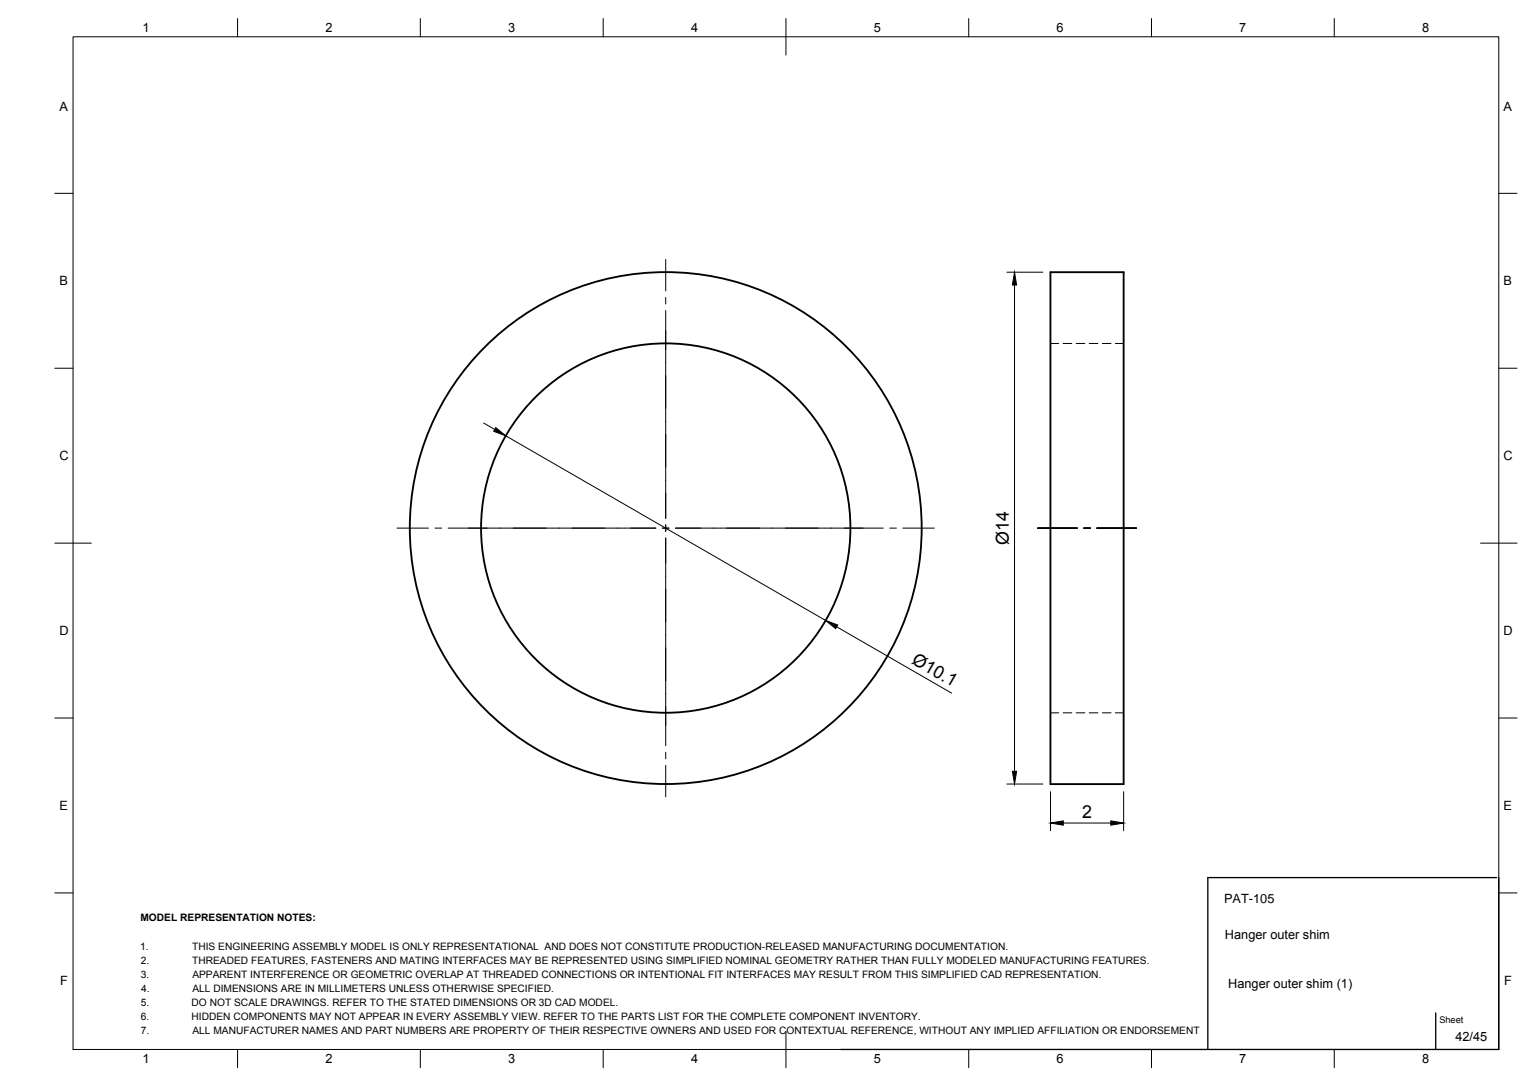
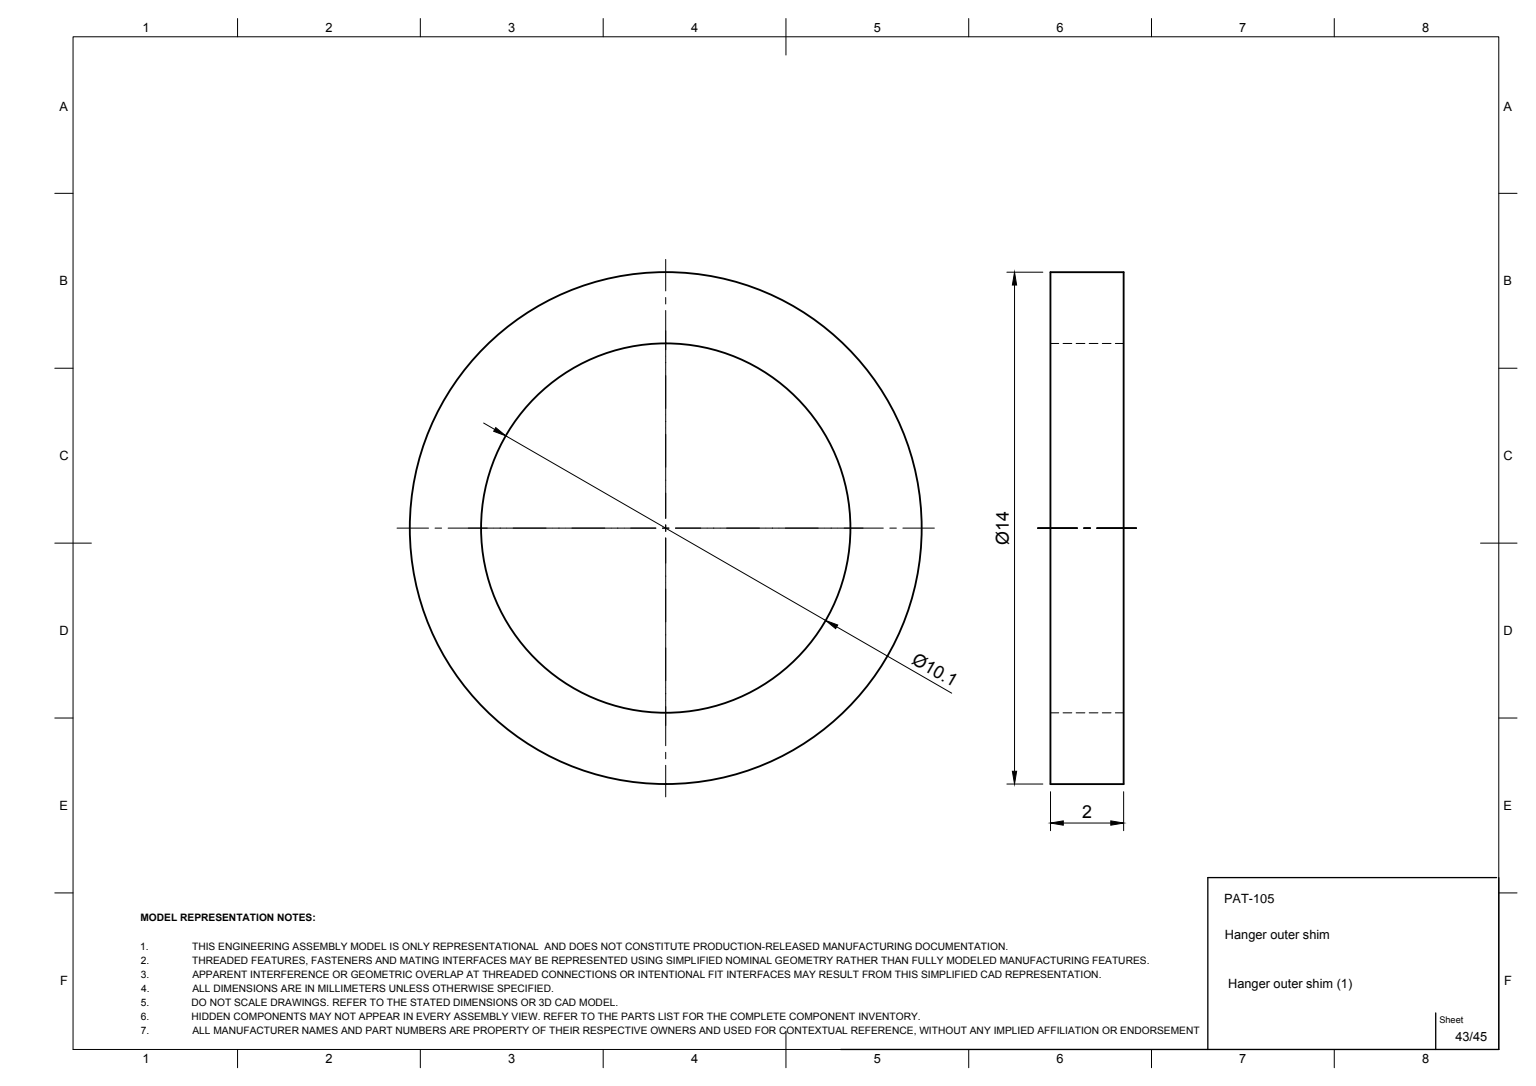
ISO-10303-21;
HEADER;
/* Generated by software containing ST-Developer
 * from STEP Tools, Inc. (www.steptools.com) 
 */

FILE_DESCRIPTION(
/* description */ ('Torque wrench calibration arm'),
/* implementation_level */ '2;1');

FILE_NAME(
/* name */ 'Hanger outer shim.step',
/* time_stamp */ '2026-10-28T03:24:52-07:00',
/* author */ (''),
/* organization */ (''),
/* preprocessor_version */ 'ST-DEVELOPER v20.2',
/* originating_system */ 'Autodesk Translation Framework v15.17.0.0',
/* authorisation */ '');

FILE_SCHEMA (('AUTOMOTIVE_DESIGN { 1 0 10303 214 3 1 1 }'));
ENDSEC;

DATA;
#10=MECHANICAL_DESIGN_GEOMETRIC_PRESENTATION_REPRESENTATION('',(#475),#12783);
#384=SHAPE_REPRESENTATION_RELATIONSHIP('SRR','None',#12969,#421);
#421=ADVANCED_BREP_SHAPE_REPRESENTATION('',(#527),#12778);
#475=STYLED_ITEM('',(#13205),#527);
#527=MANIFOLD_SOLID_BREP('Body1',#6546);
#643=FACE_BOUND('',#1748,.T.);
#644=FACE_BOUND('',#1750,.T.);
#856=PLANE('',#7744);
#857=PLANE('',#7745);
#1238=FACE_OUTER_BOUND('',#1745,.T.);
#1239=FACE_OUTER_BOUND('',#1746,.T.);
#1240=FACE_OUTER_BOUND('',#1747,.T.);
#1241=FACE_OUTER_BOUND('',#1749,.T.);
#1745=EDGE_LOOP('',(#5879,#5880,#5881,#5882));
#1746=EDGE_LOOP('',(#5883,#5884,#5885,#5886));
#1747=EDGE_LOOP('',(#5887));
#1748=EDGE_LOOP('',(#5888));
#1749=EDGE_LOOP('',(#5889));
#1750=EDGE_LOOP('',(#5890));
#2170=LINE('',#12562,#2585);
#2171=LINE('',#12568,#2586);
#2585=VECTOR('',#9754,0.505000000000003);
#2586=VECTOR('',#9761,0.700000000000003);
#2948=CIRCLE('',#7739,0.505000000000003);
#2949=CIRCLE('',#7740,0.505000000000003);
#2950=CIRCLE('',#7742,0.700000000000003);
#2951=CIRCLE('',#7743,0.700000000000003);
#3498=VERTEX_POINT('',#12559);
#3499=VERTEX_POINT('',#12561);
#3500=VERTEX_POINT('',#12565);
#3501=VERTEX_POINT('',#12567);
#4297=EDGE_CURVE('',#3498,#3498,#2948,.T.);
#4298=EDGE_CURVE('',#3498,#3499,#2170,.T.);
#4299=EDGE_CURVE('',#3499,#3499,#2949,.T.);
#4300=EDGE_CURVE('',#3500,#3500,#2950,.T.);
#4301=EDGE_CURVE('',#3500,#3501,#2171,.T.);
#4302=EDGE_CURVE('',#3501,#3501,#2951,.T.);
#5879=ORIENTED_EDGE('',*,*,#4297,.F.);
#5880=ORIENTED_EDGE('',*,*,#4298,.T.);
#5881=ORIENTED_EDGE('',*,*,#4299,.T.);
#5882=ORIENTED_EDGE('',*,*,#4298,.F.);
#5883=ORIENTED_EDGE('',*,*,#4300,.F.);
#5884=ORIENTED_EDGE('',*,*,#4301,.T.);
#5885=ORIENTED_EDGE('',*,*,#4302,.T.);
#5886=ORIENTED_EDGE('',*,*,#4301,.F.);
#5887=ORIENTED_EDGE('',*,*,#4300,.T.);
#5888=ORIENTED_EDGE('',*,*,#4297,.T.);
#5889=ORIENTED_EDGE('',*,*,#4302,.F.);
#5890=ORIENTED_EDGE('',*,*,#4299,.F.);
#6090=CYLINDRICAL_SURFACE('',#7738,0.505000000000003);
#6091=CYLINDRICAL_SURFACE('',#7741,0.700000000000003);
#6463=ADVANCED_FACE('',(#1238),#6090,.F.);
#6464=ADVANCED_FACE('',(#1239),#6091,.T.);
#6465=ADVANCED_FACE('',(#1240,#643),#856,.T.);
#6466=ADVANCED_FACE('',(#1241,#644),#857,.F.);
#6546=CLOSED_SHELL('',(#6463,#6464,#6465,#6466));
#7737=AXIS2_PLACEMENT_3D('',#12557,#9748,#9749);
#7738=AXIS2_PLACEMENT_3D('',#12558,#9750,#9751);
#7739=AXIS2_PLACEMENT_3D('',#12560,#9752,#9753);
#7740=AXIS2_PLACEMENT_3D('',#12563,#9755,#9756);
#7741=AXIS2_PLACEMENT_3D('',#12564,#9757,#9758);
#7742=AXIS2_PLACEMENT_3D('',#12566,#9759,#9760);
#7743=AXIS2_PLACEMENT_3D('',#12569,#9762,#9763);
#7744=AXIS2_PLACEMENT_3D('',#12570,#9764,#9765);
#7745=AXIS2_PLACEMENT_3D('',#12571,#9766,#9767);
#9748=DIRECTION('axis',(0.,0.,1.));
#9749=DIRECTION('refdir',(1.,0.,0.));
#9750=DIRECTION('center_axis',(0.,1.,0.));
#9751=DIRECTION('ref_axis',(1.,0.,0.));
#9752=DIRECTION('center_axis',(0.,-1.,0.));
#9753=DIRECTION('ref_axis',(1.,0.,0.));
#9754=DIRECTION('',(0.,-1.,0.));
#9755=DIRECTION('center_axis',(0.,-1.,0.));
#9756=DIRECTION('ref_axis',(1.,0.,0.));
#9757=DIRECTION('center_axis',(0.,1.,0.));
#9758=DIRECTION('ref_axis',(1.,0.,0.));
#9759=DIRECTION('center_axis',(0.,1.,0.));
#9760=DIRECTION('ref_axis',(1.,0.,0.));
#9761=DIRECTION('',(0.,-1.,0.));
#9762=DIRECTION('center_axis',(0.,1.,0.));
#9763=DIRECTION('ref_axis',(1.,0.,0.));
#9764=DIRECTION('center_axis',(0.,1.,0.));
#9765=DIRECTION('ref_axis',(1.,0.,0.));
#9766=DIRECTION('center_axis',(0.,1.,0.));
#9767=DIRECTION('ref_axis',(1.,0.,0.));
#12557=CARTESIAN_POINT('',(0.,0.,0.));
#12558=CARTESIAN_POINT('Origin',(50.,6.6,8.));
#12559=CARTESIAN_POINT('',(49.495,6.8,8.));
#12560=CARTESIAN_POINT('Origin',(50.,6.8,8.));
#12561=CARTESIAN_POINT('',(49.495,6.6,8.));
#12562=CARTESIAN_POINT('',(49.495,6.6,8.));
#12563=CARTESIAN_POINT('Origin',(50.,6.6,8.));
#12564=CARTESIAN_POINT('Origin',(50.,6.6,8.));
#12565=CARTESIAN_POINT('',(49.3,6.8,8.));
#12566=CARTESIAN_POINT('Origin',(50.,6.8,8.));
#12567=CARTESIAN_POINT('',(49.3,6.6,8.));
#12568=CARTESIAN_POINT('',(49.3,6.6,8.));
#12569=CARTESIAN_POINT('Origin',(50.,6.6,8.));
#12570=CARTESIAN_POINT('Origin',(50.,6.8,8.));
#12571=CARTESIAN_POINT('Origin',(50.,6.6,8.));
#12734=UNCERTAINTY_MEASURE_WITH_UNIT(LENGTH_MEASURE(0.001),#12784,
'DISTANCE_ACCURACY_VALUE',
'Maximum model space distance between geometric entities at asserted c
onnectivities');
#12739=UNCERTAINTY_MEASURE_WITH_UNIT(LENGTH_MEASURE(0.001),#12784,
'DISTANCE_ACCURACY_VALUE',
'Maximum model space distance between geometric entities at asserted c
onnectivities');
#12778=(
GEOMETRIC_REPRESENTATION_CONTEXT(3)
GLOBAL_UNCERTAINTY_ASSIGNED_CONTEXT((#12734))
GLOBAL_UNIT_ASSIGNED_CONTEXT((#12784,#12786,#12787))
REPRESENTATION_CONTEXT('','3D')
);
#12783=(
GEOMETRIC_REPRESENTATION_CONTEXT(3)
GLOBAL_UNCERTAINTY_ASSIGNED_CONTEXT((#12739))
GLOBAL_UNIT_ASSIGNED_CONTEXT((#12784,#12786,#12787))
REPRESENTATION_CONTEXT('','3D')
);
#12784=(
LENGTH_UNIT()
NAMED_UNIT(*)
SI_UNIT(.CENTI.,.METRE.)
);
#12786=(
NAMED_UNIT(*)
PLANE_ANGLE_UNIT()
SI_UNIT($,.RADIAN.)
);
#12787=(
NAMED_UNIT(*)
SI_UNIT($,.STERADIAN.)
SOLID_ANGLE_UNIT()
);
#12826=SHAPE_DEFINITION_REPRESENTATION(#12913,#12969);
#12913=PRODUCT_DEFINITION_SHAPE('',$,#13013);
#12969=SHAPE_REPRESENTATION('',(#7737),#12778);
#12974=PRODUCT_DEFINITION_CONTEXT('part definition',#13105,'design');
#13013=PRODUCT_DEFINITION('Hanger outer shim','Hanger outer shim',#13056,
#12974);
#13056=PRODUCT_DEFINITION_FORMATION('',$,#13145);
#13105=APPLICATION_CONTEXT(
'Core Data for Automotive Mechanical Design Process');
#13106=PRODUCT_CONTEXT('part definition',#13105,'mechanical');
#13145=PRODUCT('Hanger outer shim','Hanger outer shim',
'Hanger outer shim',(#13106));
#13199=COLOUR_RGB('Sky Blue',0.24,0.69,0.87);
#13200=FILL_AREA_STYLE_COLOUR('',#13199);
#13201=FILL_AREA_STYLE('',(#13200));
#13202=SURFACE_STYLE_FILL_AREA(#13201);
#13203=SURFACE_SIDE_STYLE('',(#13202));
#13204=SURFACE_STYLE_USAGE(.BOTH.,#13203);
#13205=PRESENTATION_STYLE_ASSIGNMENT((#13204));
ENDSEC;
END-ISO-10303-21;
